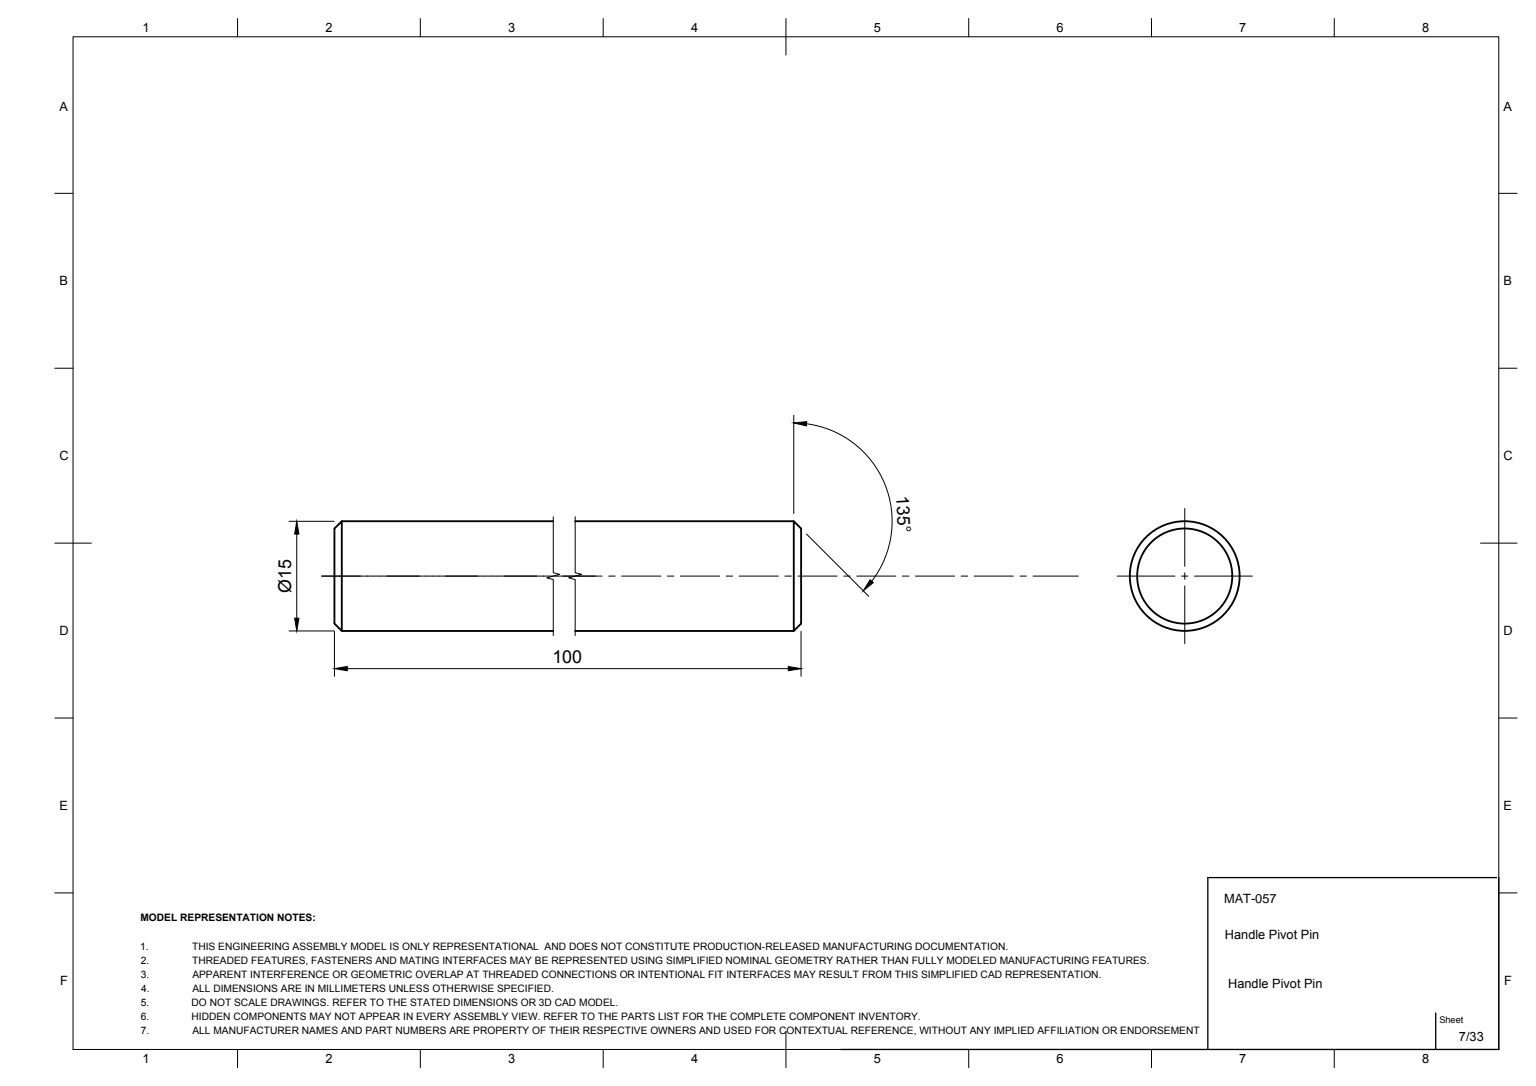
ISO-10303-21;
HEADER;
/* Generated by software containing ST-Developer
 * from STEP Tools, Inc. (www.steptools.com) 
 */

FILE_DESCRIPTION(
/* description */ ('STEP AP214', 'CAx-IF Rec.Pracs.---Representation and Presentation of Product Manufa
cturing Information (PMI)---4.0---2014-10-13'),
/* implementation_level */ '2;1');

FILE_NAME(
/* name */ 'Handle Pivot Pin.step',
/* time_stamp */ '2026-10-28T23:34:22+01:00',
/* author */ (''),
/* organization */ (''),
/* preprocessor_version */ 'ST-DEVELOPER v20.2',
/* originating_system */ 'Autodesk Translation Framework v15.17.0.0',
/* authorisation */ '');

FILE_SCHEMA (('AP242_MANAGED_MODEL_BASED_3D_ENGINEERING_MIM_LF { 1 0 10303 442 2 1 4 }'));
ENDSEC;

DATA;
#10=MECHANICAL_DESIGN_GEOMETRIC_PRESENTATION_REPRESENTATION('',(#278),#27807);
#227=SHAPE_REPRESENTATION_RELATIONSHIP('SRR','None',#27926,#249);
#249=ADVANCED_BREP_SHAPE_REPRESENTATION('',(#307),#27806);
#278=STYLED_ITEM('',(#28077),#307);
#307=MANIFOLD_SOLID_BREP('Body1',#12054);
#745=PLANE('',#13717);
#746=PLANE('',#13718);
#1246=CYLINDRICAL_SURFACE('',#13716,7.50000000000001);
#1939=FACE_OUTER_BOUND('',#2749,.T.);
#1940=FACE_OUTER_BOUND('',#2750,.T.);
#1941=FACE_OUTER_BOUND('',#2751,.T.);
#1942=FACE_OUTER_BOUND('',#2752,.T.);
#1943=FACE_OUTER_BOUND('',#2753,.T.);
#2749=EDGE_LOOP('',(#11261,#11262,#11263,#11264));
#2750=EDGE_LOOP('',(#11265,#11266,#11267,#11268,#11269));
#2751=EDGE_LOOP('',(#11270,#11271,#11272,#11273,#11274));
#2752=EDGE_LOOP('',(#11275));
#2753=EDGE_LOOP('',(#11276));
#3571=LINE('',#27723,#4391);
#3572=LINE('',#27731,#4392);
#3573=LINE('',#27734,#4393);
#4391=VECTOR('',#17375,6.49999999999999);
#4392=VECTOR('',#17384,7.50000000000001);
#4393=VECTOR('',#17389,7.50000000000001);
#5030=CIRCLE('',#13710,7.50000000000001);
#5031=CIRCLE('',#13711,6.49999999999999);
#5032=CIRCLE('',#13713,7.50000000000001);
#5033=CIRCLE('',#13714,7.50000000000001);
#5034=CIRCLE('',#13715,6.50000000000003);
#6133=VERTEX_POINT('',#27720);
#6134=VERTEX_POINT('',#27722);
#6135=VERTEX_POINT('',#27726);
#6136=VERTEX_POINT('',#27727);
#6137=VERTEX_POINT('',#27730);
#7843=EDGE_CURVE('',#6133,#6133,#5030,.T.);
#7844=EDGE_CURVE('',#6133,#6134,#3571,.T.);
#7845=EDGE_CURVE('',#6134,#6134,#5031,.T.);
#7846=EDGE_CURVE('',#6135,#6136,#5032,.T.);
#7847=EDGE_CURVE('',#6136,#6135,#5033,.T.);
#7848=EDGE_CURVE('',#6136,#6137,#3572,.T.);
#7849=EDGE_CURVE('',#6137,#6137,#5034,.T.);
#7850=EDGE_CURVE('',#6135,#6133,#3573,.T.);
#11261=ORIENTED_EDGE('',*,*,#7843,.F.);
#11262=ORIENTED_EDGE('',*,*,#7844,.T.);
#11263=ORIENTED_EDGE('',*,*,#7845,.F.);
#11264=ORIENTED_EDGE('',*,*,#7844,.F.);
#11265=ORIENTED_EDGE('',*,*,#7846,.F.);
#11266=ORIENTED_EDGE('',*,*,#7847,.F.);
#11267=ORIENTED_EDGE('',*,*,#7848,.T.);
#11268=ORIENTED_EDGE('',*,*,#7849,.F.);
#11269=ORIENTED_EDGE('',*,*,#7848,.F.);
#11270=ORIENTED_EDGE('',*,*,#7846,.T.);
#11271=ORIENTED_EDGE('',*,*,#7847,.T.);
#11272=ORIENTED_EDGE('',*,*,#7850,.T.);
#11273=ORIENTED_EDGE('',*,*,#7843,.T.);
#11274=ORIENTED_EDGE('',*,*,#7850,.F.);
#11275=ORIENTED_EDGE('',*,*,#7845,.T.);
#11276=ORIENTED_EDGE('',*,*,#7849,.T.);
#11327=CONICAL_SURFACE('',#13709,6.49999999999999,0.785398163397442);
#11328=CONICAL_SURFACE('',#13712,7.50000000000001,0.785398163397452);
#12021=ADVANCED_FACE('',(#1939),#11327,.T.);
#12022=ADVANCED_FACE('',(#1940),#11328,.T.);
#12023=ADVANCED_FACE('',(#1941),#1246,.T.);
#12024=ADVANCED_FACE('',(#1942),#745,.T.);
#12025=ADVANCED_FACE('',(#1943),#746,.F.);
#12054=CLOSED_SHELL('',(#12021,#12022,#12023,#12024,#12025));
#13708=AXIS2_PLACEMENT_3D('',#27718,#17369,#17370);
#13709=AXIS2_PLACEMENT_3D('',#27719,#17371,#17372);
#13710=AXIS2_PLACEMENT_3D('',#27721,#17373,#17374);
#13711=AXIS2_PLACEMENT_3D('',#27724,#17376,#17377);
#13712=AXIS2_PLACEMENT_3D('',#27725,#17378,#17379);
#13713=AXIS2_PLACEMENT_3D('',#27728,#17380,#17381);
#13714=AXIS2_PLACEMENT_3D('',#27729,#17382,#17383);
#13715=AXIS2_PLACEMENT_3D('',#27732,#17385,#17386);
#13716=AXIS2_PLACEMENT_3D('',#27733,#17387,#17388);
#13717=AXIS2_PLACEMENT_3D('',#27735,#17390,#17391);
#13718=AXIS2_PLACEMENT_3D('',#27736,#17392,#17393);
#17369=DIRECTION('axis',(0.,0.,1.));
#17370=DIRECTION('refdir',(1.,0.,0.));
#17371=DIRECTION('center_axis',(0.,0.,-1.));
#17372=DIRECTION('ref_axis',(-0.922798177671698,0.385283691954116,0.));
#17373=DIRECTION('center_axis',(0.,0.,-1.));
#17374=DIRECTION('ref_axis',(0.922798177671697,-0.385283691954117,0.));
#17375=DIRECTION('',(-0.652516849098242,0.272436711261342,0.707106781186552));
#17376=DIRECTION('center_axis',(0.,0.,1.));
#17377=DIRECTION('ref_axis',(0.922798177671698,-0.385283691954116,0.));
#17378=DIRECTION('center_axis',(0.,0.,1.));
#17379=DIRECTION('ref_axis',(0.922798177671697,-0.385283691954117,0.));
#17380=DIRECTION('center_axis',(0.,0.,1.));
#17381=DIRECTION('ref_axis',(0.922798177671697,-0.385283691954117,0.));
#17382=DIRECTION('center_axis',(0.,0.,1.));
#17383=DIRECTION('ref_axis',(0.922798177671697,-0.385283691954117,0.));
#17384=DIRECTION('',(0.652516849098248,-0.272436711261346,-0.707106781186545));
#17385=DIRECTION('center_axis',(0.,0.,-1.));
#17386=DIRECTION('ref_axis',(0.9227981776717,-0.385283691954111,0.));
#17387=DIRECTION('center_axis',(0.,0.,-1.));
#17388=DIRECTION('ref_axis',(-0.922798177671697,0.385283691954117,0.));
#17389=DIRECTION('',(0.,0.,1.));
#17390=DIRECTION('center_axis',(0.,0.,1.));
#17391=DIRECTION('ref_axis',(0.922798177671697,-0.385283691954116,0.));
#17392=DIRECTION('center_axis',(0.,0.,1.));
#17393=DIRECTION('ref_axis',(0.922798177671697,-0.385283691954116,0.));
#27718=CARTESIAN_POINT('',(0.,0.,0.));
#27719=CARTESIAN_POINT('Origin',(277.041252647846,78.7397376070391,303.073593133701));
#27720=CARTESIAN_POINT('',(283.962238980384,75.8501099173832,302.073593133701));
#27721=CARTESIAN_POINT('Origin',(277.041252647846,78.7397376070391,302.073593133701));
#27722=CARTESIAN_POINT('',(283.039440802712,76.2353936093374,303.073593133701));
#27723=CARTESIAN_POINT('',(283.039440802712,76.2353936093374,303.073593133701));
#27724=CARTESIAN_POINT('Origin',(277.041252647846,78.7397376070391,303.073593133701));
#27725=CARTESIAN_POINT('Origin',(277.041252647846,78.7397376070391,204.073593133701));
#27726=CARTESIAN_POINT('',(283.962238980384,75.8501099173832,204.073593133701));
#27727=CARTESIAN_POINT('',(270.120266315309,81.629365296695,204.073593133701));
#27728=CARTESIAN_POINT('Origin',(277.041252647846,78.7397376070391,204.073593133701));
#27729=CARTESIAN_POINT('Origin',(277.041252647846,78.7397376070391,204.073593133701));
#27730=CARTESIAN_POINT('',(271.04306449298,81.2440816047409,203.073593133701));
#27731=CARTESIAN_POINT('',(270.120266315309,81.629365296695,204.073593133701));
#27732=CARTESIAN_POINT('Origin',(277.041252647846,78.7397376070391,203.073593133701));
#27733=CARTESIAN_POINT('Origin',(277.041252647846,78.7397376070391,303.073593133701));
#27734=CARTESIAN_POINT('',(283.962238980384,75.8501099173832,303.073593133701));
#27735=CARTESIAN_POINT('Origin',(277.041252647846,78.7397376070391,303.073593133701));
#27736=CARTESIAN_POINT('Origin',(277.041252647846,78.7397376070391,203.073593133701));
#27777=UNCERTAINTY_MEASURE_WITH_UNIT(LENGTH_MEASURE(0.01),#27808,
'DISTANCE_ACCURACY_VALUE',
'Maximum model space distance between geometric entities at asserted c
onnectivities');
#27778=UNCERTAINTY_MEASURE_WITH_UNIT(LENGTH_MEASURE(0.01),#27808,
'DISTANCE_ACCURACY_VALUE',
'Maximum model space distance between geometric entities at asserted c
onnectivities');
#27806=(
GEOMETRIC_REPRESENTATION_CONTEXT(3)
GLOBAL_UNCERTAINTY_ASSIGNED_CONTEXT((#27777))
GLOBAL_UNIT_ASSIGNED_CONTEXT((#27808,#27810,#27811))
REPRESENTATION_CONTEXT('','3D')
);
#27807=(
GEOMETRIC_REPRESENTATION_CONTEXT(3)
GLOBAL_UNCERTAINTY_ASSIGNED_CONTEXT((#27778))
GLOBAL_UNIT_ASSIGNED_CONTEXT((#27808,#27810,#27811))
REPRESENTATION_CONTEXT('','3D')
);
#27808=(
LENGTH_UNIT()
NAMED_UNIT(*)
SI_UNIT(.MILLI.,.METRE.)
);
#27810=(
NAMED_UNIT(*)
PLANE_ANGLE_UNIT()
SI_UNIT($,.RADIAN.)
);
#27811=(
NAMED_UNIT(*)
SI_UNIT($,.STERADIAN.)
SOLID_ANGLE_UNIT()
);
#27839=SHAPE_DEFINITION_REPRESENTATION(#27885,#27926);
#27885=PRODUCT_DEFINITION_SHAPE('',$,#27955);
#27926=SHAPE_REPRESENTATION('',(#13708),#27806);
#27927=PRODUCT_DEFINITION_CONTEXT('part definition',#28013,'design');
#27955=PRODUCT_DEFINITION('Handle Pivot Pin','Handle Pivot Pin',#27983,
#27927);
#27983=PRODUCT_DEFINITION_FORMATION('',$,#28042);
#28013=APPLICATION_CONTEXT('Managed model based 3d engineering');
#28014=PRODUCT_CONTEXT('part definition',#28013,'mechanical');
#28042=PRODUCT('Handle Pivot Pin','Handle Pivot Pin',$,(#28014));
#28071=COLOUR_RGB('Grey',0.48,0.52,0.57);
#28072=FILL_AREA_STYLE_COLOUR('',#28071);
#28073=FILL_AREA_STYLE('',(#28072));
#28074=SURFACE_STYLE_FILL_AREA(#28073);
#28075=SURFACE_SIDE_STYLE('',(#28074));
#28076=SURFACE_STYLE_USAGE(.BOTH.,#28075);
#28077=PRESENTATION_STYLE_ASSIGNMENT((#28076));
ENDSEC;
END-ISO-10303-21;
